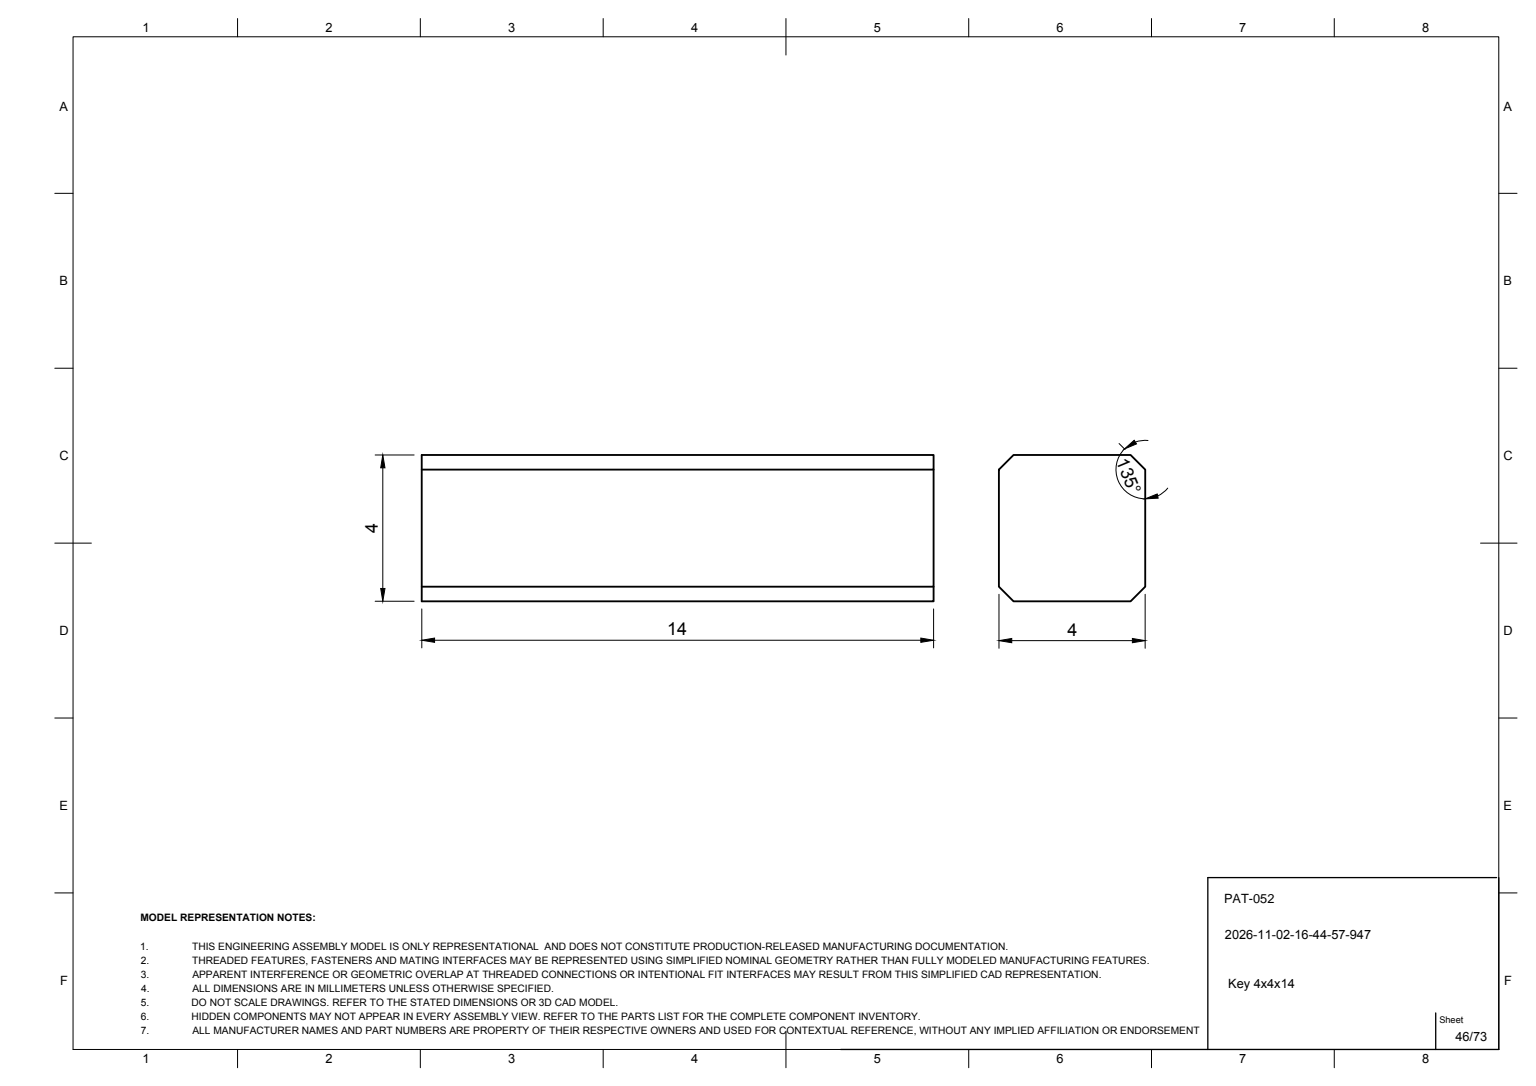
ISO-10303-21;
HEADER;
/* Generated by software containing ST-Developer
 * from STEP Tools, Inc. (www.steptools.com) 
 */

FILE_DESCRIPTION(
/* description */ ('Hand-crank gear train demonstrator'),
/* implementation_level */ '2;1');

FILE_NAME(
/* name */ 'Key 4x4x14.step',
/* time_stamp */ '2026-10-28T03:22:13-07:00',
/* author */ (''),
/* organization */ (''),
/* preprocessor_version */ 'ST-DEVELOPER v20.2',
/* originating_system */ 'Autodesk Translation Framework v15.17.0.0',
/* authorisation */ '');

FILE_SCHEMA (('AUTOMOTIVE_DESIGN { 1 0 10303 214 3 1 1 }'));
ENDSEC;

DATA;
#10=MECHANICAL_DESIGN_GEOMETRIC_PRESENTATION_REPRESENTATION('',(#1254),#62758);
#1111=SHAPE_REPRESENTATION_RELATIONSHIP('SRR','None',#63088,#1175);
#1175=ADVANCED_BREP_SHAPE_REPRESENTATION('',(#1329),#62742);
#1254=STYLED_ITEM('',(#63462),#1329);
#1329=MANIFOLD_SOLID_BREP('Body1',#16438);
#2003=PLANE('',#18365);
#2004=PLANE('',#18366);
#2005=PLANE('',#18367);
#2006=PLANE('',#18368);
#2007=PLANE('',#18369);
#2008=PLANE('',#18370);
#2009=PLANE('',#18371);
#2010=PLANE('',#18372);
#2011=PLANE('',#18373);
#2012=PLANE('',#18374);
#2786=FACE_OUTER_BOUND('',#3983,.T.);
#2787=FACE_OUTER_BOUND('',#3984,.T.);
#2788=FACE_OUTER_BOUND('',#3985,.T.);
#2789=FACE_OUTER_BOUND('',#3986,.T.);
#2790=FACE_OUTER_BOUND('',#3987,.T.);
#2791=FACE_OUTER_BOUND('',#3988,.T.);
#2792=FACE_OUTER_BOUND('',#3989,.T.);
#2793=FACE_OUTER_BOUND('',#3990,.T.);
#2794=FACE_OUTER_BOUND('',#3991,.T.);
#2795=FACE_OUTER_BOUND('',#3992,.T.);
#3983=EDGE_LOOP('',(#13765,#13766,#13767,#13768,#13769,#13770,#13771,#13772));
#3984=EDGE_LOOP('',(#13773,#13774,#13775,#13776));
#3985=EDGE_LOOP('',(#13777,#13778,#13779,#13780));
#3986=EDGE_LOOP('',(#13781,#13782,#13783,#13784));
#3987=EDGE_LOOP('',(#13785,#13786,#13787,#13788));
#3988=EDGE_LOOP('',(#13789,#13790,#13791,#13792,#13793,#13794,#13795,#13796));
#3989=EDGE_LOOP('',(#13797,#13798,#13799,#13800));
#3990=EDGE_LOOP('',(#13801,#13802,#13803,#13804));
#3991=EDGE_LOOP('',(#13805,#13806,#13807,#13808));
#3992=EDGE_LOOP('',(#13809,#13810,#13811,#13812));
#5111=LINE('',#38375,#6243);
#5112=LINE('',#38377,#6244);
#5113=LINE('',#38379,#6245);
#5114=LINE('',#38381,#6246);
#5115=LINE('',#38383,#6247);
#5116=LINE('',#38385,#6248);
#5117=LINE('',#38387,#6249);
#5118=LINE('',#38388,#6250);
#5119=LINE('',#38391,#6251);
#5120=LINE('',#38393,#6252);
#5121=LINE('',#38394,#6253);
#5122=LINE('',#38397,#6254);
#5123=LINE('',#38398,#6255);
#5124=LINE('',#38401,#6256);
#5125=LINE('',#38402,#6257);
#5126=LINE('',#38405,#6258);
#5127=LINE('',#38406,#6259);
#5128=LINE('',#38409,#6260);
#5129=LINE('',#38411,#6261);
#5130=LINE('',#38413,#6262);
#5131=LINE('',#38414,#6263);
#5132=LINE('',#38416,#6264);
#5133=LINE('',#38418,#6265);
#5134=LINE('',#38420,#6266);
#6243=VECTOR('',#22072,1.);
#6244=VECTOR('',#22073,1.);
#6245=VECTOR('',#22074,1.);
#6246=VECTOR('',#22075,1.);
#6247=VECTOR('',#22076,1.);
#6248=VECTOR('',#22077,1.);
#6249=VECTOR('',#22078,1.);
#6250=VECTOR('',#22079,1.);
#6251=VECTOR('',#22082,1.);
#6252=VECTOR('',#22083,1.);
#6253=VECTOR('',#22084,1.);
#6254=VECTOR('',#22087,1.);
#6255=VECTOR('',#22088,1.);
#6256=VECTOR('',#22091,1.);
#6257=VECTOR('',#22092,1.);
#6258=VECTOR('',#22095,1.);
#6259=VECTOR('',#22096,1.);
#6260=VECTOR('',#22099,1.);
#6261=VECTOR('',#22100,1.);
#6262=VECTOR('',#22101,1.);
#6263=VECTOR('',#22102,1.);
#6264=VECTOR('',#22105,1.);
#6265=VECTOR('',#22108,1.);
#6266=VECTOR('',#22111,1.);
#8203=VERTEX_POINT('',#38373);
#8204=VERTEX_POINT('',#38374);
#8205=VERTEX_POINT('',#38376);
#8206=VERTEX_POINT('',#38378);
#8207=VERTEX_POINT('',#38380);
#8208=VERTEX_POINT('',#38382);
#8209=VERTEX_POINT('',#38384);
#8210=VERTEX_POINT('',#38386);
#8211=VERTEX_POINT('',#38390);
#8212=VERTEX_POINT('',#38392);
#8213=VERTEX_POINT('',#38396);
#8214=VERTEX_POINT('',#38400);
#8215=VERTEX_POINT('',#38404);
#8216=VERTEX_POINT('',#38408);
#8217=VERTEX_POINT('',#38410);
#8218=VERTEX_POINT('',#38412);
#10134=EDGE_CURVE('',#8203,#8204,#5111,.T.);
#10135=EDGE_CURVE('',#8205,#8203,#5112,.T.);
#10136=EDGE_CURVE('',#8206,#8205,#5113,.T.);
#10137=EDGE_CURVE('',#8207,#8206,#5114,.T.);
#10138=EDGE_CURVE('',#8208,#8207,#5115,.T.);
#10139=EDGE_CURVE('',#8209,#8208,#5116,.T.);
#10140=EDGE_CURVE('',#8210,#8209,#5117,.T.);
#10141=EDGE_CURVE('',#8204,#8210,#5118,.T.);
#10142=EDGE_CURVE('',#8207,#8211,#5119,.T.);
#10143=EDGE_CURVE('',#8211,#8212,#5120,.T.);
#10144=EDGE_CURVE('',#8212,#8208,#5121,.T.);
#10145=EDGE_CURVE('',#8213,#8206,#5122,.T.);
#10146=EDGE_CURVE('',#8213,#8211,#5123,.T.);
#10147=EDGE_CURVE('',#8205,#8214,#5124,.T.);
#10148=EDGE_CURVE('',#8214,#8213,#5125,.T.);
#10149=EDGE_CURVE('',#8215,#8203,#5126,.T.);
#10150=EDGE_CURVE('',#8215,#8214,#5127,.T.);
#10151=EDGE_CURVE('',#8216,#8215,#5128,.T.);
#10152=EDGE_CURVE('',#8217,#8216,#5129,.T.);
#10153=EDGE_CURVE('',#8218,#8217,#5130,.T.);
#10154=EDGE_CURVE('',#8212,#8218,#5131,.T.);
#10155=EDGE_CURVE('',#8204,#8216,#5132,.T.);
#10156=EDGE_CURVE('',#8217,#8210,#5133,.T.);
#10157=EDGE_CURVE('',#8209,#8218,#5134,.T.);
#13765=ORIENTED_EDGE('',*,*,#10134,.F.);
#13766=ORIENTED_EDGE('',*,*,#10135,.F.);
#13767=ORIENTED_EDGE('',*,*,#10136,.F.);
#13768=ORIENTED_EDGE('',*,*,#10137,.F.);
#13769=ORIENTED_EDGE('',*,*,#10138,.F.);
#13770=ORIENTED_EDGE('',*,*,#10139,.F.);
#13771=ORIENTED_EDGE('',*,*,#10140,.F.);
#13772=ORIENTED_EDGE('',*,*,#10141,.F.);
#13773=ORIENTED_EDGE('',*,*,#10138,.T.);
#13774=ORIENTED_EDGE('',*,*,#10142,.T.);
#13775=ORIENTED_EDGE('',*,*,#10143,.T.);
#13776=ORIENTED_EDGE('',*,*,#10144,.T.);
#13777=ORIENTED_EDGE('',*,*,#10137,.T.);
#13778=ORIENTED_EDGE('',*,*,#10145,.F.);
#13779=ORIENTED_EDGE('',*,*,#10146,.T.);
#13780=ORIENTED_EDGE('',*,*,#10142,.F.);
#13781=ORIENTED_EDGE('',*,*,#10136,.T.);
#13782=ORIENTED_EDGE('',*,*,#10147,.T.);
#13783=ORIENTED_EDGE('',*,*,#10148,.T.);
#13784=ORIENTED_EDGE('',*,*,#10145,.T.);
#13785=ORIENTED_EDGE('',*,*,#10135,.T.);
#13786=ORIENTED_EDGE('',*,*,#10149,.F.);
#13787=ORIENTED_EDGE('',*,*,#10150,.T.);
#13788=ORIENTED_EDGE('',*,*,#10147,.F.);
#13789=ORIENTED_EDGE('',*,*,#10143,.F.);
#13790=ORIENTED_EDGE('',*,*,#10146,.F.);
#13791=ORIENTED_EDGE('',*,*,#10148,.F.);
#13792=ORIENTED_EDGE('',*,*,#10150,.F.);
#13793=ORIENTED_EDGE('',*,*,#10151,.F.);
#13794=ORIENTED_EDGE('',*,*,#10152,.F.);
#13795=ORIENTED_EDGE('',*,*,#10153,.F.);
#13796=ORIENTED_EDGE('',*,*,#10154,.F.);
#13797=ORIENTED_EDGE('',*,*,#10134,.T.);
#13798=ORIENTED_EDGE('',*,*,#10155,.T.);
#13799=ORIENTED_EDGE('',*,*,#10151,.T.);
#13800=ORIENTED_EDGE('',*,*,#10149,.T.);
#13801=ORIENTED_EDGE('',*,*,#10141,.T.);
#13802=ORIENTED_EDGE('',*,*,#10156,.F.);
#13803=ORIENTED_EDGE('',*,*,#10152,.T.);
#13804=ORIENTED_EDGE('',*,*,#10155,.F.);
#13805=ORIENTED_EDGE('',*,*,#10140,.T.);
#13806=ORIENTED_EDGE('',*,*,#10157,.T.);
#13807=ORIENTED_EDGE('',*,*,#10153,.T.);
#13808=ORIENTED_EDGE('',*,*,#10156,.T.);
#13809=ORIENTED_EDGE('',*,*,#10139,.T.);
#13810=ORIENTED_EDGE('',*,*,#10144,.F.);
#13811=ORIENTED_EDGE('',*,*,#10154,.T.);
#13812=ORIENTED_EDGE('',*,*,#10157,.F.);
#16096=ADVANCED_FACE('',(#2786),#2003,.T.);
#16097=ADVANCED_FACE('',(#2787),#2004,.T.);
#16098=ADVANCED_FACE('',(#2788),#2005,.T.);
#16099=ADVANCED_FACE('',(#2789),#2006,.T.);
#16100=ADVANCED_FACE('',(#2790),#2007,.T.);
#16101=ADVANCED_FACE('',(#2791),#2008,.F.);
#16102=ADVANCED_FACE('',(#2792),#2009,.T.);
#16103=ADVANCED_FACE('',(#2793),#2010,.T.);
#16104=ADVANCED_FACE('',(#2794),#2011,.T.);
#16105=ADVANCED_FACE('',(#2795),#2012,.F.);
#16438=CLOSED_SHELL('',(#16096,#16097,#16098,#16099,#16100,#16101,#16102,
#16103,#16104,#16105));
#18364=AXIS2_PLACEMENT_3D('',#38371,#22068,#22069);
#18365=AXIS2_PLACEMENT_3D('',#38372,#22070,#22071);
#18366=AXIS2_PLACEMENT_3D('',#38389,#22080,#22081);
#18367=AXIS2_PLACEMENT_3D('',#38395,#22085,#22086);
#18368=AXIS2_PLACEMENT_3D('',#38399,#22089,#22090);
#18369=AXIS2_PLACEMENT_3D('',#38403,#22093,#22094);
#18370=AXIS2_PLACEMENT_3D('',#38407,#22097,#22098);
#18371=AXIS2_PLACEMENT_3D('',#38415,#22103,#22104);
#18372=AXIS2_PLACEMENT_3D('',#38417,#22106,#22107);
#18373=AXIS2_PLACEMENT_3D('',#38419,#22109,#22110);
#18374=AXIS2_PLACEMENT_3D('',#38421,#22112,#22113);
#22068=DIRECTION('axis',(0.,0.,1.));
#22069=DIRECTION('refdir',(1.,0.,0.));
#22070=DIRECTION('center_axis',(1.,0.,0.));
#22071=DIRECTION('ref_axis',(0.,0.,-1.));
#22072=DIRECTION('',(0.,0.707106781186547,-0.707106781186548));
#22073=DIRECTION('',(0.,1.,0.));
#22074=DIRECTION('',(0.,0.707106781186547,0.707106781186548));
#22075=DIRECTION('',(0.,0.,1.));
#22076=DIRECTION('',(0.,-0.707106781186548,0.707106781186548));
#22077=DIRECTION('',(0.,-1.,0.));
#22078=DIRECTION('',(0.,-0.707106781186548,-0.707106781186548));
#22079=DIRECTION('',(0.,0.,-1.));
#22080=DIRECTION('center_axis',(0.,-0.707106781186548,-0.707106781186548));
#22081=DIRECTION('ref_axis',(-1.,0.,0.));
#22082=DIRECTION('',(-1.,0.,0.));
#22083=DIRECTION('',(0.,0.707106781186548,-0.707106781186548));
#22084=DIRECTION('',(1.,0.,0.));
#22085=DIRECTION('center_axis',(0.,-1.,0.));
#22086=DIRECTION('ref_axis',(1.,0.,0.));
#22087=DIRECTION('',(1.,0.,0.));
#22088=DIRECTION('',(0.,0.,-1.));
#22089=DIRECTION('center_axis',(0.,-0.707106781186548,0.707106781186547));
#22090=DIRECTION('ref_axis',(1.,0.,0.));
#22091=DIRECTION('',(-1.,0.,0.));
#22092=DIRECTION('',(0.,-0.707106781186547,-0.707106781186548));
#22093=DIRECTION('center_axis',(0.,0.,1.));
#22094=DIRECTION('ref_axis',(1.,0.,0.));
#22095=DIRECTION('',(1.,0.,0.));
#22096=DIRECTION('',(0.,-1.,0.));
#22097=DIRECTION('center_axis',(1.,0.,0.));
#22098=DIRECTION('ref_axis',(0.,0.,-1.));
#22099=DIRECTION('',(0.,-0.707106781186547,0.707106781186548));
#22100=DIRECTION('',(0.,0.,1.));
#22101=DIRECTION('',(0.,0.707106781186548,0.707106781186548));
#22102=DIRECTION('',(0.,1.,0.));
#22103=DIRECTION('center_axis',(0.,0.707106781186548,0.707106781186547));
#22104=DIRECTION('ref_axis',(1.,0.,0.));
#22105=DIRECTION('',(-1.,0.,0.));
#22106=DIRECTION('center_axis',(0.,1.,0.));
#22107=DIRECTION('ref_axis',(-1.,0.,0.));
#22108=DIRECTION('',(1.,0.,0.));
#22109=DIRECTION('center_axis',(0.,0.707106781186548,-0.707106781186548));
#22110=DIRECTION('ref_axis',(-1.,0.,0.));
#22111=DIRECTION('',(-1.,0.,0.));
#22112=DIRECTION('center_axis',(0.,0.,1.));
#22113=DIRECTION('ref_axis',(1.,0.,0.));
#38371=CARTESIAN_POINT('',(0.,0.,0.));
#38372=CARTESIAN_POINT('Origin',(0.7,0.,0.25));
#38373=CARTESIAN_POINT('',(0.7,0.16,0.4));
#38374=CARTESIAN_POINT('',(0.7,0.2,0.36));
#38375=CARTESIAN_POINT('',(0.7,0.1675,0.3925));
#38376=CARTESIAN_POINT('',(0.7,-0.16,0.4));
#38377=CARTESIAN_POINT('',(0.7,0.,0.4));
#38378=CARTESIAN_POINT('',(0.7,-0.2,0.36));
#38379=CARTESIAN_POINT('',(0.7,-0.1675,0.3925));
#38380=CARTESIAN_POINT('',(0.7,-0.2,0.04));
#38381=CARTESIAN_POINT('',(0.7,-0.2,0.125));
#38382=CARTESIAN_POINT('',(0.7,-0.16,0.));
#38383=CARTESIAN_POINT('',(0.7,-0.1925,0.0325));
#38384=CARTESIAN_POINT('',(0.7,0.16,0.));
#38385=CARTESIAN_POINT('',(0.7,0.,0.));
#38386=CARTESIAN_POINT('',(0.7,0.2,0.04));
#38387=CARTESIAN_POINT('',(0.7,0.1925,0.0325));
#38388=CARTESIAN_POINT('',(0.7,0.2,0.125));
#38389=CARTESIAN_POINT('Origin',(-0.4,-0.18,0.02));
#38390=CARTESIAN_POINT('',(-0.7,-0.2,0.04));
#38391=CARTESIAN_POINT('',(-0.4,-0.2,0.04));
#38392=CARTESIAN_POINT('',(-0.7,-0.16,0.));
#38393=CARTESIAN_POINT('',(-0.7,-0.1925,0.0325));
#38394=CARTESIAN_POINT('',(-0.4,-0.16,0.));
#38395=CARTESIAN_POINT('Origin',(-0.8,-0.2,0.));
#38396=CARTESIAN_POINT('',(-0.7,-0.2,0.36));
#38397=CARTESIAN_POINT('',(-0.4,-0.2,0.36));
#38398=CARTESIAN_POINT('',(-0.7,-0.2,0.125));
#38399=CARTESIAN_POINT('Origin',(-0.4,-0.18,0.38));
#38400=CARTESIAN_POINT('',(-0.7,-0.16,0.4));
#38401=CARTESIAN_POINT('',(-0.4,-0.16,0.4));
#38402=CARTESIAN_POINT('',(-0.7,-0.1675,0.3925));
#38403=CARTESIAN_POINT('Origin',(0.,0.,0.4));
#38404=CARTESIAN_POINT('',(-0.7,0.16,0.4));
#38405=CARTESIAN_POINT('',(0.4,0.16,0.4));
#38406=CARTESIAN_POINT('',(-0.7,0.,0.4));
#38407=CARTESIAN_POINT('Origin',(-0.7,0.,0.25));
#38408=CARTESIAN_POINT('',(-0.7,0.2,0.36));
#38409=CARTESIAN_POINT('',(-0.7,0.1675,0.3925));
#38410=CARTESIAN_POINT('',(-0.7,0.2,0.04));
#38411=CARTESIAN_POINT('',(-0.7,0.2,0.125));
#38412=CARTESIAN_POINT('',(-0.7,0.16,0.));
#38413=CARTESIAN_POINT('',(-0.7,0.1925,0.0325));
#38414=CARTESIAN_POINT('',(-0.7,0.,0.));
#38415=CARTESIAN_POINT('Origin',(0.4,0.18,0.38));
#38416=CARTESIAN_POINT('',(0.4,0.2,0.36));
#38417=CARTESIAN_POINT('Origin',(0.8,0.2,0.));
#38418=CARTESIAN_POINT('',(0.4,0.2,0.04));
#38419=CARTESIAN_POINT('Origin',(0.4,0.18,0.02));
#38420=CARTESIAN_POINT('',(0.4,0.16,0.));
#38421=CARTESIAN_POINT('Origin',(0.,0.,0.));
#62668=UNCERTAINTY_MEASURE_WITH_UNIT(LENGTH_MEASURE(0.001),#62759,
'DISTANCE_ACCURACY_VALUE',
'Maximum model space distance between geometric entities at asserted c
onnectivities');
#62684=UNCERTAINTY_MEASURE_WITH_UNIT(LENGTH_MEASURE(0.001),#62759,
'DISTANCE_ACCURACY_VALUE',
'Maximum model space distance between geometric entities at asserted c
onnectivities');
#62742=(
GEOMETRIC_REPRESENTATION_CONTEXT(3)
GLOBAL_UNCERTAINTY_ASSIGNED_CONTEXT((#62668))
GLOBAL_UNIT_ASSIGNED_CONTEXT((#62759,#62761,#62762))
REPRESENTATION_CONTEXT('','3D')
);
#62758=(
GEOMETRIC_REPRESENTATION_CONTEXT(3)
GLOBAL_UNCERTAINTY_ASSIGNED_CONTEXT((#62684))
GLOBAL_UNIT_ASSIGNED_CONTEXT((#62759,#62761,#62762))
REPRESENTATION_CONTEXT('','3D')
);
#62759=(
LENGTH_UNIT()
NAMED_UNIT(*)
SI_UNIT(.CENTI.,.METRE.)
);
#62761=(
NAMED_UNIT(*)
PLANE_ANGLE_UNIT()
SI_UNIT($,.RADIAN.)
);
#62762=(
NAMED_UNIT(*)
SI_UNIT($,.STERADIAN.)
SOLID_ANGLE_UNIT()
);
#62820=SHAPE_DEFINITION_REPRESENTATION(#62903,#63088);
#62903=PRODUCT_DEFINITION_SHAPE('',$,#63162);
#63088=SHAPE_REPRESENTATION('',(#18364),#62742);
#63104=PRODUCT_DEFINITION_CONTEXT('part definition',#63325,'design');
#63162=PRODUCT_DEFINITION('Key 4x4x14','Key 4x4x14',#63235,#63104);
#63235=PRODUCT_DEFINITION_FORMATION('',$,#63384);
#63325=APPLICATION_CONTEXT(
'Core Data for Automotive Mechanical Design Process');
#63326=PRODUCT_CONTEXT('part definition',#63325,'mechanical');
#63384=PRODUCT('Key 4x4x14','Key 4x4x14','Key 4x4x14',(#63326));
#63456=COLOUR_RGB('Grey',0.48,0.52,0.57);
#63457=FILL_AREA_STYLE_COLOUR('',#63456);
#63458=FILL_AREA_STYLE('',(#63457));
#63459=SURFACE_STYLE_FILL_AREA(#63458);
#63460=SURFACE_SIDE_STYLE('',(#63459));
#63461=SURFACE_STYLE_USAGE(.BOTH.,#63460);
#63462=PRESENTATION_STYLE_ASSIGNMENT((#63461));
ENDSEC;
END-ISO-10303-21;
